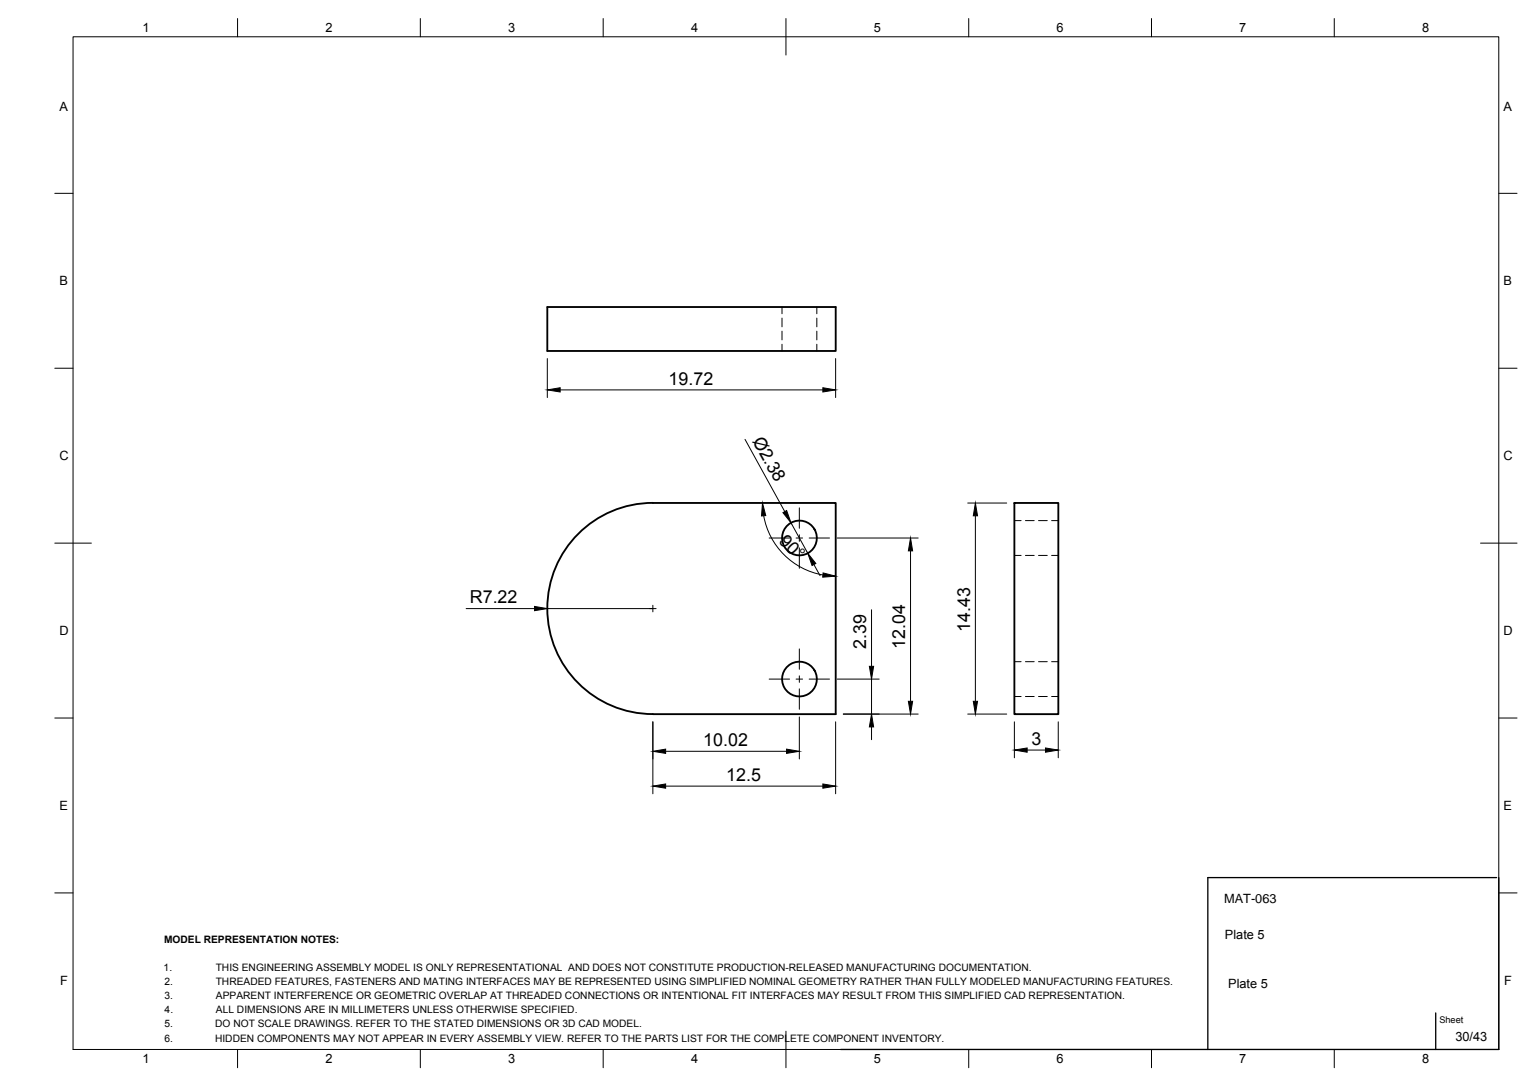
ISO-10303-21;
HEADER;
/* Generated by software containing ST-Developer
 * from STEP Tools, Inc. (www.steptools.com) 
 */

FILE_DESCRIPTION(
/* description */ (''),
/* implementation_level */ '2;1');

FILE_NAME(
/* name */ 'Plate 5.step',
/* time_stamp */ '2026-10-24T09:43:01-07:00',
/* author */ (''),
/* organization */ (''),
/* preprocessor_version */ 'ST-DEVELOPER v20.2',
/* originating_system */ 'Autodesk Translation Framework v15.15.0.0',
/* authorisation */ '');

FILE_SCHEMA (('AUTOMOTIVE_DESIGN { 1 0 10303 214 3 1 1 }'));
ENDSEC;

DATA;
#10=MECHANICAL_DESIGN_GEOMETRIC_PRESENTATION_REPRESENTATION('',(#295),#11112);
#229=SHAPE_REPRESENTATION_RELATIONSHIP('SRR','None',#11254,#262);
#262=ADVANCED_BREP_SHAPE_REPRESENTATION('',(#328),#11099);
#295=STYLED_ITEM('',(#11426),#328);
#328=MANIFOLD_SOLID_BREP('Plate 5',#6032);
#471=FACE_BOUND('',#1479,.T.);
#472=FACE_BOUND('',#1480,.T.);
#473=FACE_BOUND('',#1487,.T.);
#474=FACE_BOUND('',#1488,.T.);
#638=PLANE('',#7111);
#639=PLANE('',#7116);
#640=PLANE('',#7119);
#641=PLANE('',#7120);
#642=PLANE('',#7121);
#981=FACE_OUTER_BOUND('',#1477,.T.);
#982=FACE_OUTER_BOUND('',#1478,.T.);
#983=FACE_OUTER_BOUND('',#1481,.T.);
#984=FACE_OUTER_BOUND('',#1482,.T.);
#985=FACE_OUTER_BOUND('',#1483,.T.);
#986=FACE_OUTER_BOUND('',#1484,.T.);
#987=FACE_OUTER_BOUND('',#1485,.T.);
#988=FACE_OUTER_BOUND('',#1486,.T.);
#1477=EDGE_LOOP('',(#5293,#5294,#5295,#5296));
#1478=EDGE_LOOP('',(#5297,#5298,#5299,#5300));
#1479=EDGE_LOOP('',(#5301));
#1480=EDGE_LOOP('',(#5302));
#1481=EDGE_LOOP('',(#5303,#5304,#5305,#5306));
#1482=EDGE_LOOP('',(#5307,#5308,#5309,#5310));
#1483=EDGE_LOOP('',(#5311,#5312,#5313,#5314));
#1484=EDGE_LOOP('',(#5315,#5316,#5317,#5318));
#1485=EDGE_LOOP('',(#5319,#5320,#5321,#5322));
#1486=EDGE_LOOP('',(#5323,#5324,#5325,#5326));
#1487=EDGE_LOOP('',(#5327));
#1488=EDGE_LOOP('',(#5328));
#1868=LINE('',#10768,#2227);
#1869=LINE('',#10773,#2228);
#1870=LINE('',#10775,#2229);
#1871=LINE('',#10778,#2230);
#1872=LINE('',#10783,#2231);
#1873=LINE('',#10787,#2232);
#1874=LINE('',#10789,#2233);
#1875=LINE('',#10790,#2234);
#1876=LINE('',#10793,#2235);
#1877=LINE('',#10797,#2236);
#1878=LINE('',#10798,#2237);
#1879=LINE('',#10800,#2238);
#2227=VECTOR('',#8976,0.00118970000000007);
#2228=VECTOR('',#8981,0.01);
#2229=VECTOR('',#8982,0.01);
#2230=VECTOR('',#8985,0.01);
#2231=VECTOR('',#8990,0.00118970100000004);
#2232=VECTOR('',#8995,0.01);
#2233=VECTOR('',#8996,0.01);
#2234=VECTOR('',#8997,0.01);
#2235=VECTOR('',#9000,0.01);
#2236=VECTOR('',#9005,0.01);
#2237=VECTOR('',#9006,0.01);
#2238=VECTOR('',#9009,0.01);
#2636=CIRCLE('',#7109,0.00118970000000007);
#2637=CIRCLE('',#7110,0.00118970000000007);
#2638=CIRCLE('',#7112,0.007216878);
#2639=CIRCLE('',#7113,0.00118970100000004);
#2640=CIRCLE('',#7115,0.00118970100000004);
#2641=CIRCLE('',#7118,0.007216878);
#3110=VERTEX_POINT('',#10765);
#3111=VERTEX_POINT('',#10767);
#3112=VERTEX_POINT('',#10771);
#3113=VERTEX_POINT('',#10772);
#3114=VERTEX_POINT('',#10774);
#3115=VERTEX_POINT('',#10776);
#3116=VERTEX_POINT('',#10779);
#3117=VERTEX_POINT('',#10782);
#3118=VERTEX_POINT('',#10786);
#3119=VERTEX_POINT('',#10788);
#3120=VERTEX_POINT('',#10792);
#3121=VERTEX_POINT('',#10796);
#3850=EDGE_CURVE('',#3110,#3110,#2636,.T.);
#3851=EDGE_CURVE('',#3110,#3111,#1868,.T.);
#3852=EDGE_CURVE('',#3111,#3111,#2637,.F.);
#3853=EDGE_CURVE('',#3112,#3113,#1869,.T.);
#3854=EDGE_CURVE('',#3113,#3114,#1870,.T.);
#3855=EDGE_CURVE('',#3114,#3115,#2638,.F.);
#3856=EDGE_CURVE('',#3115,#3112,#1871,.T.);
#3857=EDGE_CURVE('',#3116,#3116,#2639,.T.);
#3858=EDGE_CURVE('',#3116,#3117,#1872,.T.);
#3859=EDGE_CURVE('',#3117,#3117,#2640,.F.);
#3860=EDGE_CURVE('',#3118,#3115,#1873,.T.);
#3861=EDGE_CURVE('',#3119,#3118,#1874,.T.);
#3862=EDGE_CURVE('',#3112,#3119,#1875,.T.);
#3863=EDGE_CURVE('',#3114,#3120,#1876,.F.);
#3864=EDGE_CURVE('',#3120,#3118,#2641,.F.);
#3865=EDGE_CURVE('',#3121,#3113,#1877,.T.);
#3866=EDGE_CURVE('',#3120,#3121,#1878,.T.);
#3867=EDGE_CURVE('',#3121,#3119,#1879,.T.);
#5293=ORIENTED_EDGE('',*,*,#3850,.F.);
#5294=ORIENTED_EDGE('',*,*,#3851,.T.);
#5295=ORIENTED_EDGE('',*,*,#3852,.F.);
#5296=ORIENTED_EDGE('',*,*,#3851,.F.);
#5297=ORIENTED_EDGE('',*,*,#3853,.T.);
#5298=ORIENTED_EDGE('',*,*,#3854,.T.);
#5299=ORIENTED_EDGE('',*,*,#3855,.T.);
#5300=ORIENTED_EDGE('',*,*,#3856,.T.);
#5301=ORIENTED_EDGE('',*,*,#3857,.T.);
#5302=ORIENTED_EDGE('',*,*,#3850,.T.);
#5303=ORIENTED_EDGE('',*,*,#3857,.F.);
#5304=ORIENTED_EDGE('',*,*,#3858,.T.);
#5305=ORIENTED_EDGE('',*,*,#3859,.F.);
#5306=ORIENTED_EDGE('',*,*,#3858,.F.);
#5307=ORIENTED_EDGE('',*,*,#3860,.F.);
#5308=ORIENTED_EDGE('',*,*,#3861,.F.);
#5309=ORIENTED_EDGE('',*,*,#3862,.F.);
#5310=ORIENTED_EDGE('',*,*,#3856,.F.);
#5311=ORIENTED_EDGE('',*,*,#3863,.T.);
#5312=ORIENTED_EDGE('',*,*,#3864,.T.);
#5313=ORIENTED_EDGE('',*,*,#3860,.T.);
#5314=ORIENTED_EDGE('',*,*,#3855,.F.);
#5315=ORIENTED_EDGE('',*,*,#3865,.F.);
#5316=ORIENTED_EDGE('',*,*,#3866,.F.);
#5317=ORIENTED_EDGE('',*,*,#3863,.F.);
#5318=ORIENTED_EDGE('',*,*,#3854,.F.);
#5319=ORIENTED_EDGE('',*,*,#3862,.T.);
#5320=ORIENTED_EDGE('',*,*,#3867,.F.);
#5321=ORIENTED_EDGE('',*,*,#3865,.T.);
#5322=ORIENTED_EDGE('',*,*,#3853,.F.);
#5323=ORIENTED_EDGE('',*,*,#3866,.T.);
#5324=ORIENTED_EDGE('',*,*,#3867,.T.);
#5325=ORIENTED_EDGE('',*,*,#3861,.T.);
#5326=ORIENTED_EDGE('',*,*,#3864,.F.);
#5327=ORIENTED_EDGE('',*,*,#3859,.T.);
#5328=ORIENTED_EDGE('',*,*,#3852,.T.);
#5617=CYLINDRICAL_SURFACE('',#7108,0.00118970000000007);
#5618=CYLINDRICAL_SURFACE('',#7114,0.00118970100000004);
#5619=CYLINDRICAL_SURFACE('',#7117,0.007216878);
#5954=ADVANCED_FACE('',(#981),#5617,.F.);
#5955=ADVANCED_FACE('',(#982,#471,#472),#638,.T.);
#5956=ADVANCED_FACE('',(#983),#5618,.F.);
#5957=ADVANCED_FACE('',(#984),#639,.F.);
#5958=ADVANCED_FACE('',(#985),#5619,.T.);
#5959=ADVANCED_FACE('',(#986),#640,.F.);
#5960=ADVANCED_FACE('',(#987),#641,.F.);
#5961=ADVANCED_FACE('',(#988,#473,#474),#642,.F.);
#6032=CLOSED_SHELL('',(#5954,#5955,#5956,#5957,#5958,#5959,#5960,#5961));
#7107=AXIS2_PLACEMENT_3D('',#10763,#8970,#8971);
#7108=AXIS2_PLACEMENT_3D('',#10764,#8972,#8973);
#7109=AXIS2_PLACEMENT_3D('',#10766,#8974,#8975);
#7110=AXIS2_PLACEMENT_3D('',#10769,#8977,#8978);
#7111=AXIS2_PLACEMENT_3D('',#10770,#8979,#8980);
#7112=AXIS2_PLACEMENT_3D('',#10777,#8983,#8984);
#7113=AXIS2_PLACEMENT_3D('',#10780,#8986,#8987);
#7114=AXIS2_PLACEMENT_3D('',#10781,#8988,#8989);
#7115=AXIS2_PLACEMENT_3D('',#10784,#8991,#8992);
#7116=AXIS2_PLACEMENT_3D('',#10785,#8993,#8994);
#7117=AXIS2_PLACEMENT_3D('',#10791,#8998,#8999);
#7118=AXIS2_PLACEMENT_3D('',#10794,#9001,#9002);
#7119=AXIS2_PLACEMENT_3D('',#10795,#9003,#9004);
#7120=AXIS2_PLACEMENT_3D('',#10799,#9007,#9008);
#7121=AXIS2_PLACEMENT_3D('',#10801,#9010,#9011);
#8970=DIRECTION('axis',(0.,0.,1.));
#8971=DIRECTION('refdir',(1.,0.,0.));
#8972=DIRECTION('center_axis',(1.,0.,0.));
#8973=DIRECTION('ref_axis',(0.,0.,-1.));
#8974=DIRECTION('center_axis',(1.,0.,0.));
#8975=DIRECTION('ref_axis',(0.,0.,-1.));
#8976=DIRECTION('',(1.,0.,0.));
#8977=DIRECTION('center_axis',(1.,0.,0.));
#8978=DIRECTION('ref_axis',(0.,0.,-1.));
#8979=DIRECTION('center_axis',(-1.,4.48048999173929E-16,8.23217897594901E-17));
#8980=DIRECTION('ref_axis',(-4.48048999173929E-16,-1.,-9.21527566961904E-49));
#8981=DIRECTION('',(4.92278448714275E-15,0.499999981040771,-0.866025414730555));
#8982=DIRECTION('',(0.,-0.866025392838329,-0.500000018959218));
#8983=DIRECTION('center_axis',(1.,0.,0.));
#8984=DIRECTION('ref_axis',(0.,0.,-1.));
#8985=DIRECTION('',(0.,0.866025412838334,0.499999984318194));
#8986=DIRECTION('center_axis',(1.,0.,0.));
#8987=DIRECTION('ref_axis',(0.,0.,-1.));
#8988=DIRECTION('center_axis',(1.,0.,0.));
#8989=DIRECTION('ref_axis',(0.,0.,-1.));
#8990=DIRECTION('',(1.,0.,0.));
#8991=DIRECTION('center_axis',(1.,0.,0.));
#8992=DIRECTION('ref_axis',(0.,0.,-1.));
#8993=DIRECTION('center_axis',(1.02825143608802E-14,0.499999984318195,-0.866025412838333));
#8994=DIRECTION('ref_axis',(1.50357456271857E-31,0.866025412838333,0.499999984318195));
#8995=DIRECTION('',(-1.,0.,0.));
#8996=DIRECTION('',(0.,-0.866025412838314,-0.499999984318228));
#8997=DIRECTION('',(1.,0.,0.));
#8998=DIRECTION('center_axis',(1.,0.,0.));
#8999=DIRECTION('ref_axis',(0.,0.,-1.));
#9000=DIRECTION('',(-1.,0.,0.));
#9001=DIRECTION('center_axis',(1.,0.,0.));
#9002=DIRECTION('ref_axis',(0.,0.,-1.));
#9003=DIRECTION('center_axis',(-4.00530144163786E-15,-0.500000018959218,
0.866025392838329));
#9004=DIRECTION('ref_axis',(1.5507230852345E-31,-0.866025392838329,-0.500000018959218));
#9005=DIRECTION('',(-1.,0.,0.));
#9006=DIRECTION('',(0.,0.866025392838324,0.500000018959226));
#9007=DIRECTION('center_axis',(6.45242124694183E-15,-0.866025414730554,
-0.499999981040772));
#9008=DIRECTION('ref_axis',(1.49042295424067E-31,0.499999981040772,-0.866025414730554));
#9009=DIRECTION('',(0.,-0.499999981040781,0.866025414730549));
#9010=DIRECTION('center_axis',(-1.,-4.77309341971722E-16,2.03395055774814E-15));
#9011=DIRECTION('ref_axis',(2.03395055774814E-15,0.,1.));
#10763=CARTESIAN_POINT('',(0.,0.,0.));
#10764=CARTESIAN_POINT('Origin',(0.477,-0.542782557,0.975695518));
#10765=CARTESIAN_POINT('',(0.477,-0.542782557,0.976885218));
#10766=CARTESIAN_POINT('Origin',(0.477,-0.542782557,0.975695518));
#10767=CARTESIAN_POINT('',(0.48,-0.542782557,0.976885218));
#10768=CARTESIAN_POINT('',(0.477,-0.542782557,0.976885218));
#10769=CARTESIAN_POINT('Origin',(0.48,-0.542782557,0.975695518));
#10770=CARTESIAN_POINT('Origin',(0.477,-0.545454380845136,0.969136388159038));
#10771=CARTESIAN_POINT('',(0.477,-0.541830423000466,0.979010345999528));
#10772=CARTESIAN_POINT('',(0.477,-0.534613544999688,0.966510345999423));
#10773=CARTESIAN_POINT('',(0.477,-0.541830422948787,0.979010345911298));
#10774=CARTESIAN_POINT('',(0.477000000016461,-0.545438861934028,0.9602603461963));
#10775=CARTESIAN_POINT('',(0.477,-0.534613545009254,0.966510345994658));
#10776=CARTESIAN_POINT('',(0.477,-0.552655740808602,0.972760345664227));
#10777=CARTESIAN_POINT('Origin',(0.477,-0.549047301,0.966510346));
#10778=CARTESIAN_POINT('',(0.477,-0.552655741001846,0.972760345998934));
#10779=CARTESIAN_POINT('',(0.477,-0.537960337,0.968532889));
#10780=CARTESIAN_POINT('Origin',(0.477,-0.537960337,0.967343188));
#10781=CARTESIAN_POINT('Origin',(0.477,-0.537960337,0.967343188));
#10782=CARTESIAN_POINT('',(0.48,-0.537960337,0.968532889));
#10783=CARTESIAN_POINT('',(0.477,-0.537960337,0.968532889));
#10784=CARTESIAN_POINT('Origin',(0.48,-0.537960337,0.967343188));
#10785=CARTESIAN_POINT('Origin',(0.4785,-0.547243082,0.975885346));
#10786=CARTESIAN_POINT('',(0.48,-0.552655740613422,0.972760345925411));
#10787=CARTESIAN_POINT('',(0.479999999999999,-0.552655741,0.972760346));
#10788=CARTESIAN_POINT('',(0.48,-0.541830423,0.979010346));
#10789=CARTESIAN_POINT('',(0.479999999999999,-0.541830423,0.979010346));
#10790=CARTESIAN_POINT('',(0.476999999999999,-0.541830423,0.979010346));
#10791=CARTESIAN_POINT('Origin',(0.477,-0.549047301,0.966510346));
#10792=CARTESIAN_POINT('',(0.48,-0.54543886200176,0.960260346156978));
#10793=CARTESIAN_POINT('',(0.47999999975,-0.545438862001176,0.960260346315308));
#10794=CARTESIAN_POINT('Origin',(0.48,-0.549047301,0.966510346));
#10795=CARTESIAN_POINT('Origin',(0.4785,-0.5400262035,0.963385346000001));
#10796=CARTESIAN_POINT('',(0.48,-0.534613545,0.966510346));
#10797=CARTESIAN_POINT('',(0.479999999999999,-0.534613545,0.966510346000001));
#10798=CARTESIAN_POINT('',(0.479999999999999,-0.545438861933347,0.960260346038483));
#10799=CARTESIAN_POINT('Origin',(0.4785,-0.538221983999999,0.972760345999999));
#10800=CARTESIAN_POINT('',(0.479999999999999,-0.534613544999999,0.966510346));
#10801=CARTESIAN_POINT('Origin',(0.48,-0.545454380845136,0.969136388159038));
#11060=UNCERTAINTY_MEASURE_WITH_UNIT(LENGTH_MEASURE(1.E-5),#11113,
'DISTANCE_ACCURACY_VALUE',
'Maximum model space distance between geometric entities at asserted c
onnectivities');
#11073=UNCERTAINTY_MEASURE_WITH_UNIT(LENGTH_MEASURE(1.E-5),#11113,
'DISTANCE_ACCURACY_VALUE',
'Maximum model space distance between geometric entities at asserted c
onnectivities');
#11099=(
GEOMETRIC_REPRESENTATION_CONTEXT(3)
GLOBAL_UNCERTAINTY_ASSIGNED_CONTEXT((#11060))
GLOBAL_UNIT_ASSIGNED_CONTEXT((#11113,#11114,#11115))
REPRESENTATION_CONTEXT('','3D')
);
#11112=(
GEOMETRIC_REPRESENTATION_CONTEXT(3)
GLOBAL_UNCERTAINTY_ASSIGNED_CONTEXT((#11073))
GLOBAL_UNIT_ASSIGNED_CONTEXT((#11113,#11114,#11115))
REPRESENTATION_CONTEXT('','3D')
);
#11113=(
LENGTH_UNIT()
NAMED_UNIT(*)
SI_UNIT($,.METRE.)
);
#11114=(
NAMED_UNIT(*)
PLANE_ANGLE_UNIT()
SI_UNIT($,.RADIAN.)
);
#11115=(
NAMED_UNIT(*)
SI_UNIT($,.STERADIAN.)
SOLID_ANGLE_UNIT()
);
#11141=SHAPE_DEFINITION_REPRESENTATION(#11186,#11254);
#11186=PRODUCT_DEFINITION_SHAPE('',$,#11293);
#11254=SHAPE_REPRESENTATION('',(#7107),#11099);
#11267=PRODUCT_DEFINITION_CONTEXT('part definition',#11383,'design');
#11293=PRODUCT_DEFINITION('Plate 5','Plate 5',#11331,#11267);
#11331=PRODUCT_DEFINITION_FORMATION('',$,#11410);
#11383=APPLICATION_CONTEXT(
'Core Data for Automotive Mechanical Design Process');
#11384=PRODUCT_CONTEXT('part definition',#11383,'mechanical');
#11410=PRODUCT('Plate 5','Plate 5','all_plates__ DE     1563',(#11384));
#11426=PRESENTATION_STYLE_ASSIGNMENT((#11430));
#11430=SURFACE_STYLE_USAGE(.BOTH.,#11434);
#11434=SURFACE_SIDE_STYLE('',(#11438));
#11438=SURFACE_STYLE_FILL_AREA(#11442);
#11442=FILL_AREA_STYLE('Opaque(202,209,238)',(#11446));
#11446=FILL_AREA_STYLE_COLOUR('Opaque(202,209,238)',#11450);
#11450=COLOUR_RGB('Opaque(202,209,238)',0.792156862745098,0.819607843137255,
0.933333333333333);
ENDSEC;
END-ISO-10303-21;
